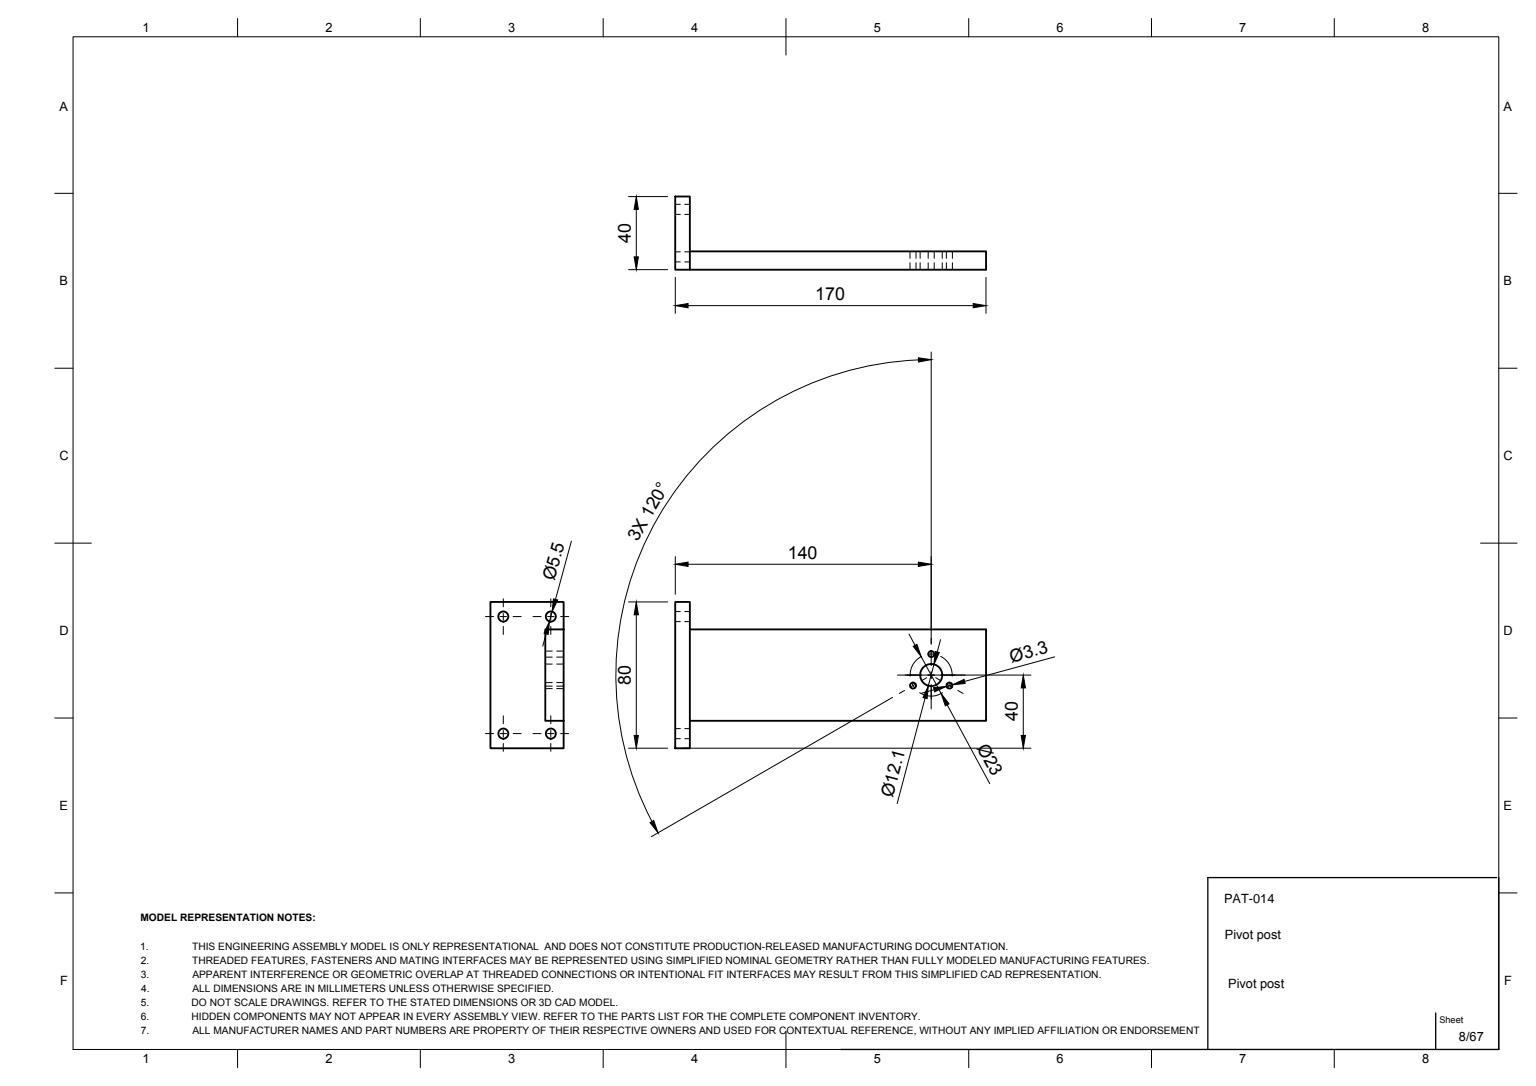
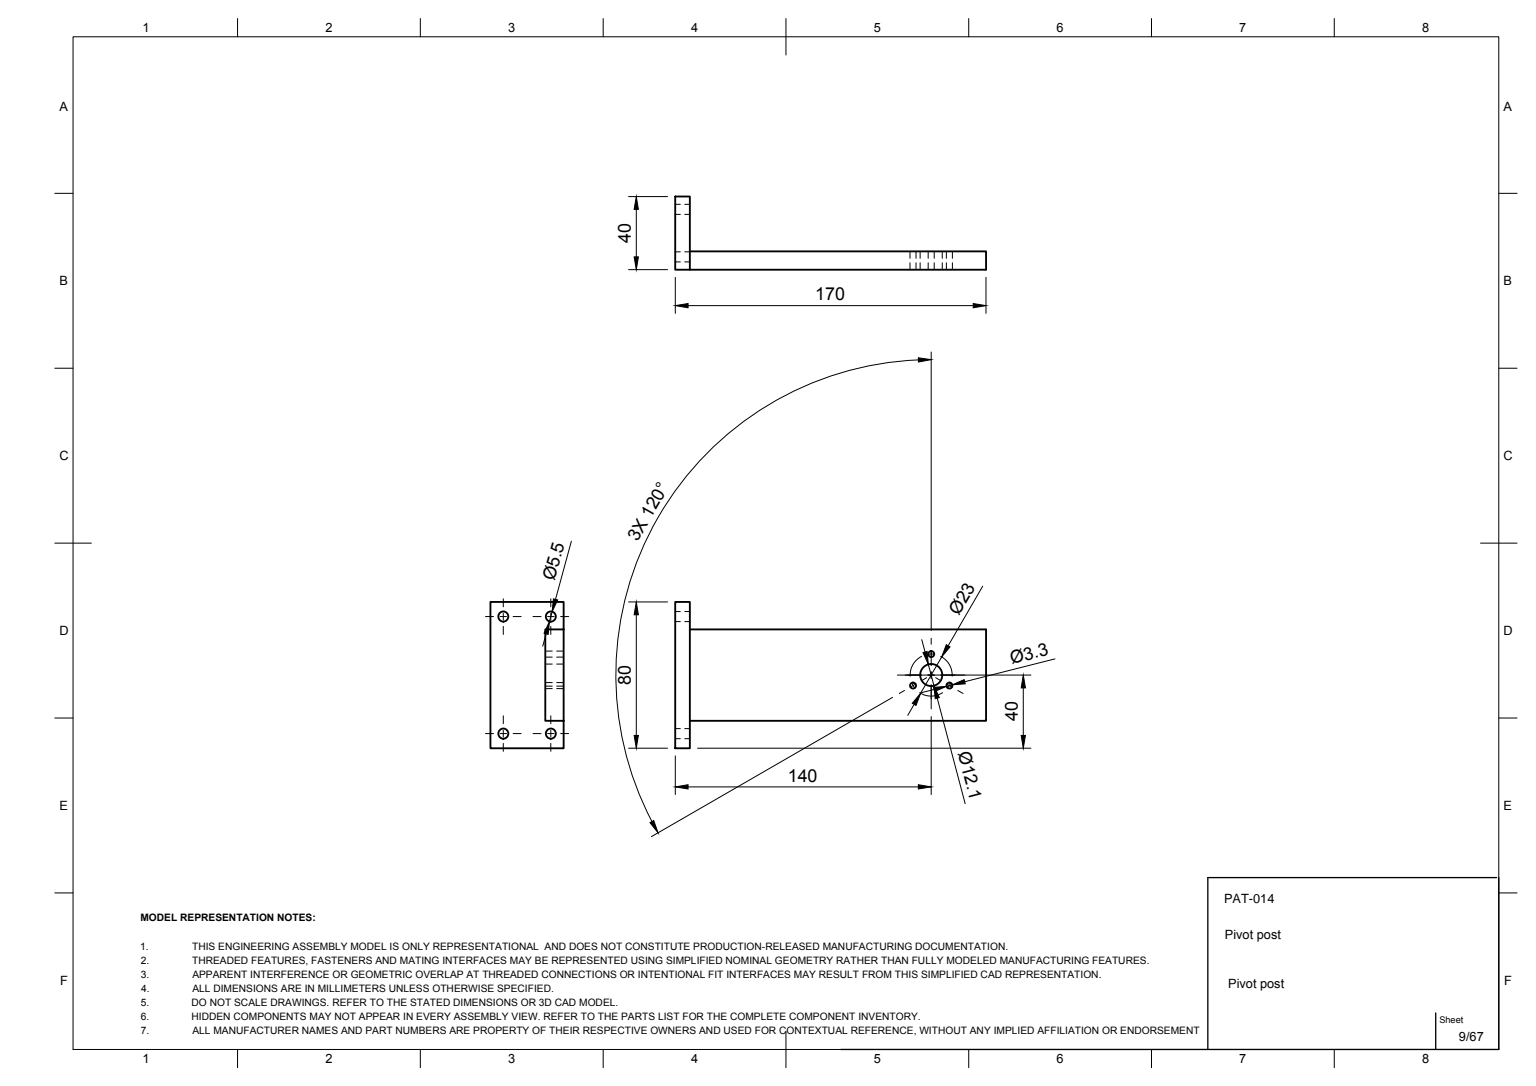
ISO-10303-21;
HEADER;
/* Generated by software containing ST-Developer
 * from STEP Tools, Inc. (www.steptools.com) 
 */

FILE_DESCRIPTION(
/* description */ ('Bin tilter linkage'),
/* implementation_level */ '2;1');

FILE_NAME(
/* name */ 'Pivot post.step',
/* time_stamp */ '2026-10-28T03:26:24-07:00',
/* author */ (''),
/* organization */ (''),
/* preprocessor_version */ 'ST-DEVELOPER v20.2',
/* originating_system */ 'Autodesk Translation Framework v15.17.0.0',
/* authorisation */ '');

FILE_SCHEMA (('AUTOMOTIVE_DESIGN { 1 0 10303 214 3 1 1 }'));
ENDSEC;

DATA;
#10=MECHANICAL_DESIGN_GEOMETRIC_PRESENTATION_REPRESENTATION('',(#865),#23728);
#653=SHAPE_REPRESENTATION_RELATIONSHIP('SRR','None',#24117,#759);
#759=ADVANCED_BREP_SHAPE_REPRESENTATION('',(#979),#23617);
#865=STYLED_ITEM('',(#24779),#979);
#979=MANIFOLD_SOLID_BREP('Body1',#12395);
#1111=FACE_BOUND('',#2730,.T.);
#1112=FACE_BOUND('',#2731,.T.);
#1113=FACE_BOUND('',#2732,.T.);
#1114=FACE_BOUND('',#2733,.T.);
#1115=FACE_BOUND('',#2738,.T.);
#1116=FACE_BOUND('',#2739,.T.);
#1117=FACE_BOUND('',#2740,.T.);
#1118=FACE_BOUND('',#2741,.T.);
#1119=FACE_BOUND('',#2744,.T.);
#1120=FACE_BOUND('',#2745,.T.);
#1121=FACE_BOUND('',#2746,.T.);
#1122=FACE_BOUND('',#2747,.T.);
#1123=FACE_BOUND('',#2751,.T.);
#1124=FACE_BOUND('',#2752,.T.);
#1125=FACE_BOUND('',#2753,.T.);
#1126=FACE_BOUND('',#2754,.T.);
#1510=PLANE('',#13760);
#1511=PLANE('',#13761);
#1512=PLANE('',#13762);
#1513=PLANE('',#13763);
#1514=PLANE('',#13764);
#1515=PLANE('',#13765);
#1516=PLANE('',#13766);
#1517=PLANE('',#13767);
#1518=PLANE('',#13768);
#1519=PLANE('',#13769);
#1920=FACE_OUTER_BOUND('',#2721,.T.);
#1921=FACE_OUTER_BOUND('',#2722,.T.);
#1922=FACE_OUTER_BOUND('',#2723,.T.);
#1923=FACE_OUTER_BOUND('',#2724,.T.);
#1924=FACE_OUTER_BOUND('',#2725,.T.);
#1925=FACE_OUTER_BOUND('',#2726,.T.);
#1926=FACE_OUTER_BOUND('',#2727,.T.);
#1927=FACE_OUTER_BOUND('',#2728,.T.);
#1928=FACE_OUTER_BOUND('',#2729,.T.);
#1929=FACE_OUTER_BOUND('',#2734,.T.);
#1930=FACE_OUTER_BOUND('',#2735,.T.);
#1931=FACE_OUTER_BOUND('',#2736,.T.);
#1932=FACE_OUTER_BOUND('',#2737,.T.);
#1933=FACE_OUTER_BOUND('',#2742,.T.);
#1934=FACE_OUTER_BOUND('',#2743,.T.);
#1935=FACE_OUTER_BOUND('',#2748,.T.);
#1936=FACE_OUTER_BOUND('',#2749,.T.);
#1937=FACE_OUTER_BOUND('',#2750,.T.);
#2721=EDGE_LOOP('',(#8517,#8518,#8519,#8520));
#2722=EDGE_LOOP('',(#8521,#8522,#8523,#8524));
#2723=EDGE_LOOP('',(#8525,#8526,#8527,#8528));
#2724=EDGE_LOOP('',(#8529,#8530,#8531,#8532));
#2725=EDGE_LOOP('',(#8533,#8534,#8535,#8536));
#2726=EDGE_LOOP('',(#8537,#8538,#8539,#8540));
#2727=EDGE_LOOP('',(#8541,#8542,#8543,#8544));
#2728=EDGE_LOOP('',(#8545,#8546,#8547,#8548));
#2729=EDGE_LOOP('',(#8549,#8550,#8551,#8552,#8553,#8554,#8555,#8556));
#2730=EDGE_LOOP('',(#8557));
#2731=EDGE_LOOP('',(#8558));
#2732=EDGE_LOOP('',(#8559));
#2733=EDGE_LOOP('',(#8560));
#2734=EDGE_LOOP('',(#8561,#8562,#8563,#8564));
#2735=EDGE_LOOP('',(#8565,#8566,#8567,#8568));
#2736=EDGE_LOOP('',(#8569,#8570,#8571,#8572));
#2737=EDGE_LOOP('',(#8573,#8574,#8575,#8576,#8577,#8578,#8579,#8580));
#2738=EDGE_LOOP('',(#8581));
#2739=EDGE_LOOP('',(#8582));
#2740=EDGE_LOOP('',(#8583));
#2741=EDGE_LOOP('',(#8584));
#2742=EDGE_LOOP('',(#8585,#8586,#8587,#8588));
#2743=EDGE_LOOP('',(#8589,#8590,#8591,#8592));
#2744=EDGE_LOOP('',(#8593));
#2745=EDGE_LOOP('',(#8594));
#2746=EDGE_LOOP('',(#8595));
#2747=EDGE_LOOP('',(#8596));
#2748=EDGE_LOOP('',(#8597,#8598,#8599,#8600));
#2749=EDGE_LOOP('',(#8601,#8602,#8603,#8604));
#2750=EDGE_LOOP('',(#8605,#8606,#8607,#8608));
#2751=EDGE_LOOP('',(#8609));
#2752=EDGE_LOOP('',(#8610));
#2753=EDGE_LOOP('',(#8611));
#2754=EDGE_LOOP('',(#8612));
#3897=LINE('',#19905,#4572);
#3898=LINE('',#19911,#4573);
#3899=LINE('',#19917,#4574);
#3900=LINE('',#19923,#4575);
#3901=LINE('',#19929,#4576);
#3902=LINE('',#19935,#4577);
#3903=LINE('',#19941,#4578);
#3904=LINE('',#19947,#4579);
#3905=LINE('',#19952,#4580);
#3906=LINE('',#19954,#4581);
#3907=LINE('',#19956,#4582);
#3908=LINE('',#19958,#4583);
#3909=LINE('',#19960,#4584);
#3910=LINE('',#19962,#4585);
#3911=LINE('',#19964,#4586);
#3912=LINE('',#19965,#4587);
#3913=LINE('',#19968,#4588);
#3914=LINE('',#19970,#4589);
#3915=LINE('',#19971,#4590);
#3916=LINE('',#19974,#4591);
#3917=LINE('',#19976,#4592);
#3918=LINE('',#19977,#4593);
#3919=LINE('',#19979,#4594);
#3920=LINE('',#19982,#4595);
#3921=LINE('',#19984,#4596);
#3922=LINE('',#19985,#4597);
#3923=LINE('',#19986,#4598);
#3924=LINE('',#19989,#4599);
#3925=LINE('',#19990,#4600);
#3926=LINE('',#19993,#4601);
#3927=LINE('',#19994,#4602);
#3928=LINE('',#19996,#4603);
#4572=VECTOR('',#15646,0.165);
#4573=VECTOR('',#15653,0.165);
#4574=VECTOR('',#15660,0.165);
#4575=VECTOR('',#15667,0.605);
#4576=VECTOR('',#15674,0.275);
#4577=VECTOR('',#15681,0.275);
#4578=VECTOR('',#15688,0.275);
#4579=VECTOR('',#15695,0.275);
#4580=VECTOR('',#15700,1.);
#4581=VECTOR('',#15701,1.);
#4582=VECTOR('',#15702,1.);
#4583=VECTOR('',#15703,1.);
#4584=VECTOR('',#15704,1.);
#4585=VECTOR('',#15705,1.);
#4586=VECTOR('',#15706,1.);
#4587=VECTOR('',#15707,1.);
#4588=VECTOR('',#15710,1.);
#4589=VECTOR('',#15711,1.);
#4590=VECTOR('',#15712,1.);
#4591=VECTOR('',#15715,1.);
#4592=VECTOR('',#15716,1.);
#4593=VECTOR('',#15717,1.);
#4594=VECTOR('',#15720,1.);
#4595=VECTOR('',#15723,1.);
#4596=VECTOR('',#15724,1.);
#4597=VECTOR('',#15725,1.);
#4598=VECTOR('',#15726,1.);
#4599=VECTOR('',#15729,1.);
#4600=VECTOR('',#15730,1.);
#4601=VECTOR('',#15733,1.);
#4602=VECTOR('',#15734,1.);
#4603=VECTOR('',#15737,1.);
#5223=CIRCLE('',#13737,0.165);
#5224=CIRCLE('',#13738,0.165);
#5225=CIRCLE('',#13740,0.165);
#5226=CIRCLE('',#13741,0.165);
#5227=CIRCLE('',#13743,0.165);
#5228=CIRCLE('',#13744,0.165);
#5229=CIRCLE('',#13746,0.605);
#5230=CIRCLE('',#13747,0.605);
#5231=CIRCLE('',#13749,0.275);
#5232=CIRCLE('',#13750,0.275);
#5233=CIRCLE('',#13752,0.275);
#5234=CIRCLE('',#13753,0.275);
#5235=CIRCLE('',#13755,0.275);
#5236=CIRCLE('',#13756,0.275);
#5237=CIRCLE('',#13758,0.275);
#5238=CIRCLE('',#13759,0.275);
#6005=VERTEX_POINT('',#19902);
#6006=VERTEX_POINT('',#19904);
#6007=VERTEX_POINT('',#19908);
#6008=VERTEX_POINT('',#19910);
#6009=VERTEX_POINT('',#19914);
#6010=VERTEX_POINT('',#19916);
#6011=VERTEX_POINT('',#19920);
#6012=VERTEX_POINT('',#19922);
#6013=VERTEX_POINT('',#19926);
#6014=VERTEX_POINT('',#19928);
#6015=VERTEX_POINT('',#19932);
#6016=VERTEX_POINT('',#19934);
#6017=VERTEX_POINT('',#19938);
#6018=VERTEX_POINT('',#19940);
#6019=VERTEX_POINT('',#19944);
#6020=VERTEX_POINT('',#19946);
#6021=VERTEX_POINT('',#19950);
#6022=VERTEX_POINT('',#19951);
#6023=VERTEX_POINT('',#19953);
#6024=VERTEX_POINT('',#19955);
#6025=VERTEX_POINT('',#19957);
#6026=VERTEX_POINT('',#19959);
#6027=VERTEX_POINT('',#19961);
#6028=VERTEX_POINT('',#19963);
#6029=VERTEX_POINT('',#19967);
#6030=VERTEX_POINT('',#19969);
#6031=VERTEX_POINT('',#19973);
#6032=VERTEX_POINT('',#19975);
#6033=VERTEX_POINT('',#19981);
#6034=VERTEX_POINT('',#19983);
#6035=VERTEX_POINT('',#19988);
#6036=VERTEX_POINT('',#19992);
#6998=EDGE_CURVE('',#6005,#6005,#5223,.T.);
#6999=EDGE_CURVE('',#6005,#6006,#3897,.T.);
#7000=EDGE_CURVE('',#6006,#6006,#5224,.T.);
#7001=EDGE_CURVE('',#6007,#6007,#5225,.T.);
#7002=EDGE_CURVE('',#6007,#6008,#3898,.T.);
#7003=EDGE_CURVE('',#6008,#6008,#5226,.T.);
#7004=EDGE_CURVE('',#6009,#6009,#5227,.T.);
#7005=EDGE_CURVE('',#6009,#6010,#3899,.T.);
#7006=EDGE_CURVE('',#6010,#6010,#5228,.T.);
#7007=EDGE_CURVE('',#6011,#6011,#5229,.T.);
#7008=EDGE_CURVE('',#6011,#6012,#3900,.T.);
#7009=EDGE_CURVE('',#6012,#6012,#5230,.T.);
#7010=EDGE_CURVE('',#6013,#6013,#5231,.T.);
#7011=EDGE_CURVE('',#6013,#6014,#3901,.T.);
#7012=EDGE_CURVE('',#6014,#6014,#5232,.T.);
#7013=EDGE_CURVE('',#6015,#6015,#5233,.T.);
#7014=EDGE_CURVE('',#6015,#6016,#3902,.T.);
#7015=EDGE_CURVE('',#6016,#6016,#5234,.T.);
#7016=EDGE_CURVE('',#6017,#6017,#5235,.T.);
#7017=EDGE_CURVE('',#6017,#6018,#3903,.T.);
#7018=EDGE_CURVE('',#6018,#6018,#5236,.T.);
#7019=EDGE_CURVE('',#6019,#6019,#5237,.T.);
#7020=EDGE_CURVE('',#6019,#6020,#3904,.T.);
#7021=EDGE_CURVE('',#6020,#6020,#5238,.T.);
#7022=EDGE_CURVE('',#6021,#6022,#3905,.T.);
#7023=EDGE_CURVE('',#6023,#6021,#3906,.T.);
#7024=EDGE_CURVE('',#6024,#6023,#3907,.T.);
#7025=EDGE_CURVE('',#6025,#6024,#3908,.T.);
#7026=EDGE_CURVE('',#6025,#6026,#3909,.T.);
#7027=EDGE_CURVE('',#6027,#6026,#3910,.T.);
#7028=EDGE_CURVE('',#6028,#6027,#3911,.T.);
#7029=EDGE_CURVE('',#6022,#6028,#3912,.T.);
#7030=EDGE_CURVE('',#6028,#6029,#3913,.T.);
#7031=EDGE_CURVE('',#6030,#6027,#3914,.T.);
#7032=EDGE_CURVE('',#6029,#6030,#3915,.T.);
#7033=EDGE_CURVE('',#6031,#6025,#3916,.T.);
#7034=EDGE_CURVE('',#6031,#6032,#3917,.T.);
#7035=EDGE_CURVE('',#6026,#6032,#3918,.T.);
#7036=EDGE_CURVE('',#6032,#6030,#3919,.T.);
#7037=EDGE_CURVE('',#6024,#6033,#3920,.T.);
#7038=EDGE_CURVE('',#6034,#6033,#3921,.T.);
#7039=EDGE_CURVE('',#6022,#6034,#3922,.T.);
#7040=EDGE_CURVE('',#6029,#6031,#3923,.T.);
#7041=EDGE_CURVE('',#6023,#6035,#3924,.T.);
#7042=EDGE_CURVE('',#6033,#6035,#3925,.T.);
#7043=EDGE_CURVE('',#6021,#6036,#3926,.T.);
#7044=EDGE_CURVE('',#6035,#6036,#3927,.T.);
#7045=EDGE_CURVE('',#6036,#6034,#3928,.T.);
#8517=ORIENTED_EDGE('',*,*,#6998,.F.);
#8518=ORIENTED_EDGE('',*,*,#6999,.T.);
#8519=ORIENTED_EDGE('',*,*,#7000,.F.);
#8520=ORIENTED_EDGE('',*,*,#6999,.F.);
#8521=ORIENTED_EDGE('',*,*,#7001,.F.);
#8522=ORIENTED_EDGE('',*,*,#7002,.T.);
#8523=ORIENTED_EDGE('',*,*,#7003,.F.);
#8524=ORIENTED_EDGE('',*,*,#7002,.F.);
#8525=ORIENTED_EDGE('',*,*,#7004,.F.);
#8526=ORIENTED_EDGE('',*,*,#7005,.T.);
#8527=ORIENTED_EDGE('',*,*,#7006,.F.);
#8528=ORIENTED_EDGE('',*,*,#7005,.F.);
#8529=ORIENTED_EDGE('',*,*,#7007,.F.);
#8530=ORIENTED_EDGE('',*,*,#7008,.T.);
#8531=ORIENTED_EDGE('',*,*,#7009,.F.);
#8532=ORIENTED_EDGE('',*,*,#7008,.F.);
#8533=ORIENTED_EDGE('',*,*,#7010,.F.);
#8534=ORIENTED_EDGE('',*,*,#7011,.T.);
#8535=ORIENTED_EDGE('',*,*,#7012,.F.);
#8536=ORIENTED_EDGE('',*,*,#7011,.F.);
#8537=ORIENTED_EDGE('',*,*,#7013,.F.);
#8538=ORIENTED_EDGE('',*,*,#7014,.T.);
#8539=ORIENTED_EDGE('',*,*,#7015,.F.);
#8540=ORIENTED_EDGE('',*,*,#7014,.F.);
#8541=ORIENTED_EDGE('',*,*,#7016,.F.);
#8542=ORIENTED_EDGE('',*,*,#7017,.T.);
#8543=ORIENTED_EDGE('',*,*,#7018,.F.);
#8544=ORIENTED_EDGE('',*,*,#7017,.F.);
#8545=ORIENTED_EDGE('',*,*,#7019,.F.);
#8546=ORIENTED_EDGE('',*,*,#7020,.T.);
#8547=ORIENTED_EDGE('',*,*,#7021,.F.);
#8548=ORIENTED_EDGE('',*,*,#7020,.F.);
#8549=ORIENTED_EDGE('',*,*,#7022,.F.);
#8550=ORIENTED_EDGE('',*,*,#7023,.F.);
#8551=ORIENTED_EDGE('',*,*,#7024,.F.);
#8552=ORIENTED_EDGE('',*,*,#7025,.F.);
#8553=ORIENTED_EDGE('',*,*,#7026,.T.);
#8554=ORIENTED_EDGE('',*,*,#7027,.F.);
#8555=ORIENTED_EDGE('',*,*,#7028,.F.);
#8556=ORIENTED_EDGE('',*,*,#7029,.F.);
#8557=ORIENTED_EDGE('',*,*,#7012,.T.);
#8558=ORIENTED_EDGE('',*,*,#7015,.T.);
#8559=ORIENTED_EDGE('',*,*,#7018,.T.);
#8560=ORIENTED_EDGE('',*,*,#7021,.T.);
#8561=ORIENTED_EDGE('',*,*,#7030,.F.);
#8562=ORIENTED_EDGE('',*,*,#7028,.T.);
#8563=ORIENTED_EDGE('',*,*,#7031,.F.);
#8564=ORIENTED_EDGE('',*,*,#7032,.F.);
#8565=ORIENTED_EDGE('',*,*,#7033,.F.);
#8566=ORIENTED_EDGE('',*,*,#7034,.T.);
#8567=ORIENTED_EDGE('',*,*,#7035,.F.);
#8568=ORIENTED_EDGE('',*,*,#7026,.F.);
#8569=ORIENTED_EDGE('',*,*,#7027,.T.);
#8570=ORIENTED_EDGE('',*,*,#7035,.T.);
#8571=ORIENTED_EDGE('',*,*,#7036,.T.);
#8572=ORIENTED_EDGE('',*,*,#7031,.T.);
#8573=ORIENTED_EDGE('',*,*,#7037,.T.);
#8574=ORIENTED_EDGE('',*,*,#7038,.F.);
#8575=ORIENTED_EDGE('',*,*,#7039,.F.);
#8576=ORIENTED_EDGE('',*,*,#7029,.T.);
#8577=ORIENTED_EDGE('',*,*,#7030,.T.);
#8578=ORIENTED_EDGE('',*,*,#7040,.T.);
#8579=ORIENTED_EDGE('',*,*,#7033,.T.);
#8580=ORIENTED_EDGE('',*,*,#7025,.T.);
#8581=ORIENTED_EDGE('',*,*,#6998,.T.);
#8582=ORIENTED_EDGE('',*,*,#7001,.T.);
#8583=ORIENTED_EDGE('',*,*,#7004,.T.);
#8584=ORIENTED_EDGE('',*,*,#7007,.T.);
#8585=ORIENTED_EDGE('',*,*,#7024,.T.);
#8586=ORIENTED_EDGE('',*,*,#7041,.T.);
#8587=ORIENTED_EDGE('',*,*,#7042,.F.);
#8588=ORIENTED_EDGE('',*,*,#7037,.F.);
#8589=ORIENTED_EDGE('',*,*,#7023,.T.);
#8590=ORIENTED_EDGE('',*,*,#7043,.T.);
#8591=ORIENTED_EDGE('',*,*,#7044,.F.);
#8592=ORIENTED_EDGE('',*,*,#7041,.F.);
#8593=ORIENTED_EDGE('',*,*,#7000,.T.);
#8594=ORIENTED_EDGE('',*,*,#7003,.T.);
#8595=ORIENTED_EDGE('',*,*,#7006,.T.);
#8596=ORIENTED_EDGE('',*,*,#7009,.T.);
#8597=ORIENTED_EDGE('',*,*,#7022,.T.);
#8598=ORIENTED_EDGE('',*,*,#7039,.T.);
#8599=ORIENTED_EDGE('',*,*,#7045,.F.);
#8600=ORIENTED_EDGE('',*,*,#7043,.F.);
#8601=ORIENTED_EDGE('',*,*,#7045,.T.);
#8602=ORIENTED_EDGE('',*,*,#7038,.T.);
#8603=ORIENTED_EDGE('',*,*,#7042,.T.);
#8604=ORIENTED_EDGE('',*,*,#7044,.T.);
#8605=ORIENTED_EDGE('',*,*,#7040,.F.);
#8606=ORIENTED_EDGE('',*,*,#7032,.T.);
#8607=ORIENTED_EDGE('',*,*,#7036,.F.);
#8608=ORIENTED_EDGE('',*,*,#7034,.F.);
#8609=ORIENTED_EDGE('',*,*,#7010,.T.);
#8610=ORIENTED_EDGE('',*,*,#7013,.T.);
#8611=ORIENTED_EDGE('',*,*,#7016,.T.);
#8612=ORIENTED_EDGE('',*,*,#7019,.T.);
#11279=CYLINDRICAL_SURFACE('',#13736,0.165);
#11280=CYLINDRICAL_SURFACE('',#13739,0.165);
#11281=CYLINDRICAL_SURFACE('',#13742,0.165);
#11282=CYLINDRICAL_SURFACE('',#13745,0.605);
#11283=CYLINDRICAL_SURFACE('',#13748,0.275);
#11284=CYLINDRICAL_SURFACE('',#13751,0.275);
#11285=CYLINDRICAL_SURFACE('',#13754,0.275);
#11286=CYLINDRICAL_SURFACE('',#13757,0.275);
#11645=ADVANCED_FACE('',(#1920),#11279,.F.);
#11646=ADVANCED_FACE('',(#1921),#11280,.F.);
#11647=ADVANCED_FACE('',(#1922),#11281,.F.);
#11648=ADVANCED_FACE('',(#1923),#11282,.F.);
#11649=ADVANCED_FACE('',(#1924),#11283,.F.);
#11650=ADVANCED_FACE('',(#1925),#11284,.F.);
#11651=ADVANCED_FACE('',(#1926),#11285,.F.);
#11652=ADVANCED_FACE('',(#1927),#11286,.F.);
#11653=ADVANCED_FACE('',(#1928,#1111,#1112,#1113,#1114),#1510,.T.);
#11654=ADVANCED_FACE('',(#1929),#1511,.T.);
#11655=ADVANCED_FACE('',(#1930),#1512,.T.);
#11656=ADVANCED_FACE('',(#1931),#1513,.T.);
#11657=ADVANCED_FACE('',(#1932,#1115,#1116,#1117,#1118),#1514,.T.);
#11658=ADVANCED_FACE('',(#1933),#1515,.T.);
#11659=ADVANCED_FACE('',(#1934,#1119,#1120,#1121,#1122),#1516,.T.);
#11660=ADVANCED_FACE('',(#1935),#1517,.T.);
#11661=ADVANCED_FACE('',(#1936),#1518,.T.);
#11662=ADVANCED_FACE('',(#1937,#1123,#1124,#1125,#1126),#1519,.F.);
#12395=CLOSED_SHELL('',(#11645,#11646,#11647,#11648,#11649,#11650,#11651,
#11652,#11653,#11654,#11655,#11656,#11657,#11658,#11659,#11660,#11661,#11662));
#13735=AXIS2_PLACEMENT_3D('',#19900,#15640,#15641);
#13736=AXIS2_PLACEMENT_3D('',#19901,#15642,#15643);
#13737=AXIS2_PLACEMENT_3D('',#19903,#15644,#15645);
#13738=AXIS2_PLACEMENT_3D('',#19906,#15647,#15648);
#13739=AXIS2_PLACEMENT_3D('',#19907,#15649,#15650);
#13740=AXIS2_PLACEMENT_3D('',#19909,#15651,#15652);
#13741=AXIS2_PLACEMENT_3D('',#19912,#15654,#15655);
#13742=AXIS2_PLACEMENT_3D('',#19913,#15656,#15657);
#13743=AXIS2_PLACEMENT_3D('',#19915,#15658,#15659);
#13744=AXIS2_PLACEMENT_3D('',#19918,#15661,#15662);
#13745=AXIS2_PLACEMENT_3D('',#19919,#15663,#15664);
#13746=AXIS2_PLACEMENT_3D('',#19921,#15665,#15666);
#13747=AXIS2_PLACEMENT_3D('',#19924,#15668,#15669);
#13748=AXIS2_PLACEMENT_3D('',#19925,#15670,#15671);
#13749=AXIS2_PLACEMENT_3D('',#19927,#15672,#15673);
#13750=AXIS2_PLACEMENT_3D('',#19930,#15675,#15676);
#13751=AXIS2_PLACEMENT_3D('',#19931,#15677,#15678);
#13752=AXIS2_PLACEMENT_3D('',#19933,#15679,#15680);
#13753=AXIS2_PLACEMENT_3D('',#19936,#15682,#15683);
#13754=AXIS2_PLACEMENT_3D('',#19937,#15684,#15685);
#13755=AXIS2_PLACEMENT_3D('',#19939,#15686,#15687);
#13756=AXIS2_PLACEMENT_3D('',#19942,#15689,#15690);
#13757=AXIS2_PLACEMENT_3D('',#19943,#15691,#15692);
#13758=AXIS2_PLACEMENT_3D('',#19945,#15693,#15694);
#13759=AXIS2_PLACEMENT_3D('',#19948,#15696,#15697);
#13760=AXIS2_PLACEMENT_3D('',#19949,#15698,#15699);
#13761=AXIS2_PLACEMENT_3D('',#19966,#15708,#15709);
#13762=AXIS2_PLACEMENT_3D('',#19972,#15713,#15714);
#13763=AXIS2_PLACEMENT_3D('',#19978,#15718,#15719);
#13764=AXIS2_PLACEMENT_3D('',#19980,#15721,#15722);
#13765=AXIS2_PLACEMENT_3D('',#19987,#15727,#15728);
#13766=AXIS2_PLACEMENT_3D('',#19991,#15731,#15732);
#13767=AXIS2_PLACEMENT_3D('',#19995,#15735,#15736);
#13768=AXIS2_PLACEMENT_3D('',#19997,#15738,#15739);
#13769=AXIS2_PLACEMENT_3D('',#19998,#15740,#15741);
#15640=DIRECTION('axis',(0.,0.,1.));
#15641=DIRECTION('refdir',(1.,0.,0.));
#15642=DIRECTION('center_axis',(0.,1.,0.));
#15643=DIRECTION('ref_axis',(1.,0.,0.));
#15644=DIRECTION('center_axis',(0.,1.,0.));
#15645=DIRECTION('ref_axis',(1.,0.,0.));
#15646=DIRECTION('',(0.,1.,0.));
#15647=DIRECTION('center_axis',(0.,-1.,0.));
#15648=DIRECTION('ref_axis',(1.,0.,0.));
#15649=DIRECTION('center_axis',(0.,1.,0.));
#15650=DIRECTION('ref_axis',(1.,0.,0.));
#15651=DIRECTION('center_axis',(0.,1.,0.));
#15652=DIRECTION('ref_axis',(1.,0.,0.));
#15653=DIRECTION('',(0.,1.,0.));
#15654=DIRECTION('center_axis',(0.,-1.,0.));
#15655=DIRECTION('ref_axis',(1.,0.,0.));
#15656=DIRECTION('center_axis',(0.,1.,0.));
#15657=DIRECTION('ref_axis',(1.,0.,0.));
#15658=DIRECTION('center_axis',(0.,1.,0.));
#15659=DIRECTION('ref_axis',(1.,0.,0.));
#15660=DIRECTION('',(0.,1.,0.));
#15661=DIRECTION('center_axis',(0.,-1.,0.));
#15662=DIRECTION('ref_axis',(1.,0.,0.));
#15663=DIRECTION('center_axis',(0.,1.,0.));
#15664=DIRECTION('ref_axis',(1.,0.,0.));
#15665=DIRECTION('center_axis',(0.,1.,0.));
#15666=DIRECTION('ref_axis',(1.,0.,0.));
#15667=DIRECTION('',(0.,1.,0.));
#15668=DIRECTION('center_axis',(0.,-1.,0.));
#15669=DIRECTION('ref_axis',(1.,0.,0.));
#15670=DIRECTION('center_axis',(0.,0.,1.));
#15671=DIRECTION('ref_axis',(1.,0.,0.));
#15672=DIRECTION('center_axis',(0.,0.,1.));
#15673=DIRECTION('ref_axis',(1.,0.,0.));
#15674=DIRECTION('',(0.,0.,1.));
#15675=DIRECTION('center_axis',(0.,0.,-1.));
#15676=DIRECTION('ref_axis',(1.,0.,0.));
#15677=DIRECTION('center_axis',(0.,0.,1.));
#15678=DIRECTION('ref_axis',(1.,0.,0.));
#15679=DIRECTION('center_axis',(0.,0.,1.));
#15680=DIRECTION('ref_axis',(1.,0.,0.));
#15681=DIRECTION('',(0.,0.,1.));
#15682=DIRECTION('center_axis',(0.,0.,-1.));
#15683=DIRECTION('ref_axis',(1.,0.,0.));
#15684=DIRECTION('center_axis',(0.,0.,1.));
#15685=DIRECTION('ref_axis',(1.,0.,0.));
#15686=DIRECTION('center_axis',(0.,0.,1.));
#15687=DIRECTION('ref_axis',(1.,0.,0.));
#15688=DIRECTION('',(0.,0.,1.));
#15689=DIRECTION('center_axis',(0.,0.,-1.));
#15690=DIRECTION('ref_axis',(1.,0.,0.));
#15691=DIRECTION('center_axis',(0.,0.,1.));
#15692=DIRECTION('ref_axis',(1.,0.,0.));
#15693=DIRECTION('center_axis',(0.,0.,1.));
#15694=DIRECTION('ref_axis',(1.,0.,0.));
#15695=DIRECTION('',(0.,0.,1.));
#15696=DIRECTION('center_axis',(0.,0.,-1.));
#15697=DIRECTION('ref_axis',(1.,0.,0.));
#15698=DIRECTION('center_axis',(0.,0.,1.));
#15699=DIRECTION('ref_axis',(1.,0.,0.));
#15700=DIRECTION('',(0.,-1.,0.));
#15701=DIRECTION('',(-1.,0.,0.));
#15702=DIRECTION('',(0.,1.,0.));
#15703=DIRECTION('',(-1.,0.,0.));
#15704=DIRECTION('',(0.,1.,0.));
#15705=DIRECTION('',(1.,0.,0.));
#15706=DIRECTION('',(0.,1.,0.));
#15707=DIRECTION('',(-1.,0.,0.));
#15708=DIRECTION('center_axis',(-1.,0.,0.));
#15709=DIRECTION('ref_axis',(0.,0.,1.));
#15710=DIRECTION('',(0.,0.,-1.));
#15711=DIRECTION('',(0.,0.,1.));
#15712=DIRECTION('',(0.,1.,0.));
#15713=DIRECTION('center_axis',(1.,0.,0.));
#15714=DIRECTION('ref_axis',(0.,0.,-1.));
#15715=DIRECTION('',(0.,0.,1.));
#15716=DIRECTION('',(0.,1.,0.));
#15717=DIRECTION('',(0.,0.,-1.));
#15718=DIRECTION('center_axis',(0.,1.,0.));
#15719=DIRECTION('ref_axis',(0.,0.,1.));
#15720=DIRECTION('',(-1.,0.,0.));
#15721=DIRECTION('center_axis',(0.,-1.,0.));
#15722=DIRECTION('ref_axis',(1.,0.,0.));
#15723=DIRECTION('',(0.,0.,1.));
#15724=DIRECTION('',(1.,0.,0.));
#15725=DIRECTION('',(0.,0.,1.));
#15726=DIRECTION('',(1.,0.,0.));
#15727=DIRECTION('center_axis',(1.,0.,0.));
#15728=DIRECTION('ref_axis',(0.,1.,0.));
#15729=DIRECTION('',(0.,0.,1.));
#15730=DIRECTION('',(0.,1.,0.));
#15731=DIRECTION('center_axis',(0.,1.,0.));
#15732=DIRECTION('ref_axis',(-1.,0.,0.));
#15733=DIRECTION('',(0.,0.,1.));
#15734=DIRECTION('',(-1.,0.,0.));
#15735=DIRECTION('center_axis',(-1.,0.,0.));
#15736=DIRECTION('ref_axis',(0.,-1.,0.));
#15737=DIRECTION('',(0.,-1.,0.));
#15738=DIRECTION('center_axis',(0.,0.,1.));
#15739=DIRECTION('ref_axis',(1.,0.,0.));
#15740=DIRECTION('center_axis',(0.,0.,1.));
#15741=DIRECTION('ref_axis',(1.,0.,0.));
#19900=CARTESIAN_POINT('',(0.,0.,0.));
#19901=CARTESIAN_POINT('Origin',(1.15,4.4,15.));
#19902=CARTESIAN_POINT('',(0.985,4.5,15.));
#19903=CARTESIAN_POINT('Origin',(1.15,4.5,15.));
#19904=CARTESIAN_POINT('',(0.985,5.5,15.));
#19905=CARTESIAN_POINT('',(0.985,4.4,15.));
#19906=CARTESIAN_POINT('Origin',(1.15,5.5,15.));
#19907=CARTESIAN_POINT('Origin',(-0.575,4.4,15.9959292143521));
#19908=CARTESIAN_POINT('',(-0.74,4.5,15.9959292143521));
#19909=CARTESIAN_POINT('Origin',(-0.575,4.5,15.9959292143521));
#19910=CARTESIAN_POINT('',(-0.74,5.5,15.9959292143521));
#19911=CARTESIAN_POINT('',(-0.74,4.4,15.9959292143521));
#19912=CARTESIAN_POINT('Origin',(-0.575,5.5,15.9959292143521));
#19913=CARTESIAN_POINT('Origin',(-0.575000000000001,4.4,14.0040707856479));
#19914=CARTESIAN_POINT('',(-0.74,4.5,14.0040707856479));
#19915=CARTESIAN_POINT('Origin',(-0.575000000000001,4.5,14.0040707856479));
#19916=CARTESIAN_POINT('',(-0.74,5.5,14.0040707856479));
#19917=CARTESIAN_POINT('',(-0.74,4.4,14.0040707856479));
#19918=CARTESIAN_POINT('Origin',(-0.575000000000001,5.5,14.0040707856479));
#19919=CARTESIAN_POINT('Origin',(0.,4.4,15.));
#19920=CARTESIAN_POINT('',(-0.605,4.5,15.));
#19921=CARTESIAN_POINT('Origin',(0.,4.5,15.));
#19922=CARTESIAN_POINT('',(-0.605,5.5,15.));
#19923=CARTESIAN_POINT('',(-0.605,4.4,15.));
#19924=CARTESIAN_POINT('Origin',(0.,5.5,15.));
#19925=CARTESIAN_POINT('Origin',(3.2,7.8,0.9));
#19926=CARTESIAN_POINT('',(2.925,7.8,1.));
#19927=CARTESIAN_POINT('Origin',(3.2,7.8,1.));
#19928=CARTESIAN_POINT('',(2.925,7.8,1.8));
#19929=CARTESIAN_POINT('',(2.925,7.8,0.9));
#19930=CARTESIAN_POINT('Origin',(3.2,7.8,1.8));
#19931=CARTESIAN_POINT('Origin',(3.2,5.2,0.9));
#19932=CARTESIAN_POINT('',(2.925,5.2,1.));
#19933=CARTESIAN_POINT('Origin',(3.2,5.2,1.));
#19934=CARTESIAN_POINT('',(2.925,5.2,1.8));
#19935=CARTESIAN_POINT('',(2.925,5.2,0.9));
#19936=CARTESIAN_POINT('Origin',(3.2,5.2,1.8));
#19937=CARTESIAN_POINT('Origin',(-3.2,7.8,0.9));
#19938=CARTESIAN_POINT('',(-3.475,7.8,1.));
#19939=CARTESIAN_POINT('Origin',(-3.2,7.8,1.));
#19940=CARTESIAN_POINT('',(-3.475,7.8,1.8));
#19941=CARTESIAN_POINT('',(-3.475,7.8,0.9));
#19942=CARTESIAN_POINT('Origin',(-3.2,7.8,1.8));
#19943=CARTESIAN_POINT('Origin',(-3.2,5.2,0.9));
#19944=CARTESIAN_POINT('',(-3.475,5.2,1.));
#19945=CARTESIAN_POINT('Origin',(-3.2,5.2,1.));
#19946=CARTESIAN_POINT('',(-3.475,5.2,1.8));
#19947=CARTESIAN_POINT('',(-3.475,5.2,0.9));
#19948=CARTESIAN_POINT('Origin',(-3.2,5.2,1.8));
#19949=CARTESIAN_POINT('Origin',(-4.,4.5,1.8));
#19950=CARTESIAN_POINT('',(-2.5,5.5,1.8));
#19951=CARTESIAN_POINT('',(-2.5,4.5,1.8));
#19952=CARTESIAN_POINT('',(-2.5,5.,1.8));
#19953=CARTESIAN_POINT('',(2.5,5.5,1.8));
#19954=CARTESIAN_POINT('',(-0.75,5.5,1.8));
#19955=CARTESIAN_POINT('',(2.5,4.5,1.8));
#19956=CARTESIAN_POINT('',(2.5,4.5,1.8));
#19957=CARTESIAN_POINT('',(4.,4.5,1.8));
#19958=CARTESIAN_POINT('',(4.,4.5,1.8));
#19959=CARTESIAN_POINT('',(4.,8.5,1.8));
#19960=CARTESIAN_POINT('',(4.,4.5,1.8));
#19961=CARTESIAN_POINT('',(-4.,8.5,1.8));
#19962=CARTESIAN_POINT('',(4.,8.5,1.8));
#19963=CARTESIAN_POINT('',(-4.,4.5,1.8));
#19964=CARTESIAN_POINT('',(-4.,4.5,1.8));
#19965=CARTESIAN_POINT('',(4.,4.5,1.8));
#19966=CARTESIAN_POINT('Origin',(-4.,4.5,1.));
#19967=CARTESIAN_POINT('',(-4.,4.5,1.));
#19968=CARTESIAN_POINT('',(-4.,4.5,1.8));
#19969=CARTESIAN_POINT('',(-4.,8.5,1.));
#19970=CARTESIAN_POINT('',(-4.,8.5,1.8));
#19971=CARTESIAN_POINT('',(-4.,4.5,1.));
#19972=CARTESIAN_POINT('Origin',(4.,4.5,1.8));
#19973=CARTESIAN_POINT('',(4.,4.5,1.));
#19974=CARTESIAN_POINT('',(4.,4.5,1.));
#19975=CARTESIAN_POINT('',(4.,8.5,1.));
#19976=CARTESIAN_POINT('',(4.,4.5,1.));
#19977=CARTESIAN_POINT('',(4.,8.5,1.));
#19978=CARTESIAN_POINT('Origin',(0.,8.5,1.4));
#19979=CARTESIAN_POINT('',(-4.,8.5,1.));
#19980=CARTESIAN_POINT('Origin',(-2.5,4.5,1.));
#19981=CARTESIAN_POINT('',(2.5,4.5,18.));
#19982=CARTESIAN_POINT('',(2.5,4.5,1.));
#19983=CARTESIAN_POINT('',(-2.5,4.5,18.));
#19984=CARTESIAN_POINT('',(-2.5,4.5,18.));
#19985=CARTESIAN_POINT('',(-2.5,4.5,1.));
#19986=CARTESIAN_POINT('',(-4.,4.5,1.));
#19987=CARTESIAN_POINT('Origin',(2.5,4.5,1.));
#19988=CARTESIAN_POINT('',(2.5,5.5,18.));
#19989=CARTESIAN_POINT('',(2.5,5.5,1.));
#19990=CARTESIAN_POINT('',(2.5,4.5,18.));
#19991=CARTESIAN_POINT('Origin',(2.5,5.5,1.));
#19992=CARTESIAN_POINT('',(-2.5,5.5,18.));
#19993=CARTESIAN_POINT('',(-2.5,5.5,1.));
#19994=CARTESIAN_POINT('',(2.5,5.5,18.));
#19995=CARTESIAN_POINT('Origin',(-2.5,5.5,1.));
#19996=CARTESIAN_POINT('',(-2.5,5.5,18.));
#19997=CARTESIAN_POINT('Origin',(0.,5.,18.));
#19998=CARTESIAN_POINT('Origin',(0.,5.,1.));
#23500=UNCERTAINTY_MEASURE_WITH_UNIT(LENGTH_MEASURE(0.001),#23729,
'DISTANCE_ACCURACY_VALUE',
'Maximum model space distance between geometric entities at asserted c
onnectivities');
#23611=UNCERTAINTY_MEASURE_WITH_UNIT(LENGTH_MEASURE(0.001),#23729,
'DISTANCE_ACCURACY_VALUE',
'Maximum model space distance between geometric entities at asserted c
onnectivities');
#23617=(
GEOMETRIC_REPRESENTATION_CONTEXT(3)
GLOBAL_UNCERTAINTY_ASSIGNED_CONTEXT((#23500))
GLOBAL_UNIT_ASSIGNED_CONTEXT((#23729,#23731,#23732))
REPRESENTATION_CONTEXT('','3D')
);
#23728=(
GEOMETRIC_REPRESENTATION_CONTEXT(3)
GLOBAL_UNCERTAINTY_ASSIGNED_CONTEXT((#23611))
GLOBAL_UNIT_ASSIGNED_CONTEXT((#23729,#23731,#23732))
REPRESENTATION_CONTEXT('','3D')
);
#23729=(
LENGTH_UNIT()
NAMED_UNIT(*)
SI_UNIT(.CENTI.,.METRE.)
);
#23731=(
NAMED_UNIT(*)
PLANE_ANGLE_UNIT()
SI_UNIT($,.RADIAN.)
);
#23732=(
NAMED_UNIT(*)
SI_UNIT($,.STERADIAN.)
SOLID_ANGLE_UNIT()
);
#23738=SHAPE_DEFINITION_REPRESENTATION(#23854,#24117);
#23854=PRODUCT_DEFINITION_SHAPE('',$,#24234);
#24117=SHAPE_REPRESENTATION('',(#13735),#23617);
#24228=PRODUCT_DEFINITION_CONTEXT('part definition',#24578,'design');
#24234=PRODUCT_DEFINITION('Pivot post','Pivot post',#24350,#24228);
#24350=PRODUCT_DEFINITION_FORMATION('',$,#24585);
#24578=APPLICATION_CONTEXT(
'Core Data for Automotive Mechanical Design Process');
#24579=PRODUCT_CONTEXT('part definition',#24578,'mechanical');
#24585=PRODUCT('Pivot post','Pivot post','Pivot post',(#24579));
#24773=COLOUR_RGB('Off White',0.89,0.88,0.83);
#24774=FILL_AREA_STYLE_COLOUR('',#24773);
#24775=FILL_AREA_STYLE('',(#24774));
#24776=SURFACE_STYLE_FILL_AREA(#24775);
#24777=SURFACE_SIDE_STYLE('',(#24776));
#24778=SURFACE_STYLE_USAGE(.BOTH.,#24777);
#24779=PRESENTATION_STYLE_ASSIGNMENT((#24778));
ENDSEC;
END-ISO-10303-21;
